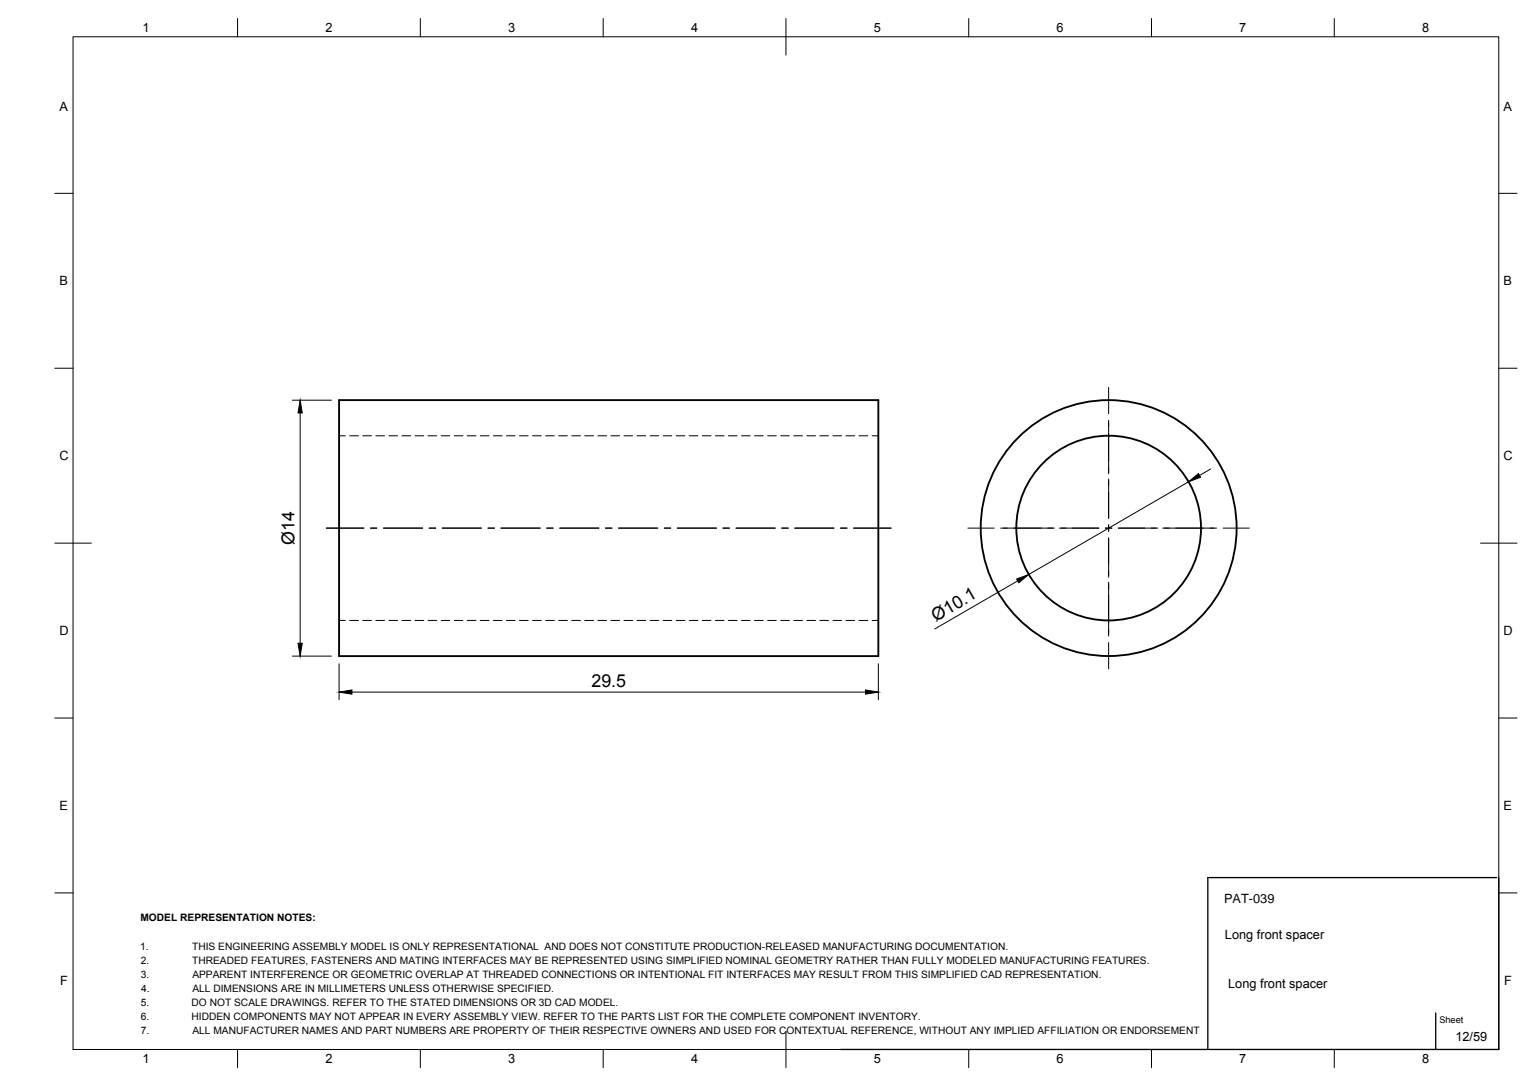
ISO-10303-21;
HEADER;
/* Generated by software containing ST-Developer
 * from STEP Tools, Inc. (www.steptools.com) 
 */

FILE_DESCRIPTION(
/* description */ ('Four-bar parallelogram arm'),
/* implementation_level */ '2;1');

FILE_NAME(
/* name */ 'Long front spacer.step',
/* time_stamp */ '2026-10-28T03:24:55-07:00',
/* author */ (''),
/* organization */ (''),
/* preprocessor_version */ 'ST-DEVELOPER v20.2',
/* originating_system */ 'Autodesk Translation Framework v15.17.0.0',
/* authorisation */ '');

FILE_SCHEMA (('AUTOMOTIVE_DESIGN { 1 0 10303 214 3 1 1 }'));
ENDSEC;

DATA;
#10=MECHANICAL_DESIGN_GEOMETRIC_PRESENTATION_REPRESENTATION('',(#629),#14512);
#529=SHAPE_REPRESENTATION_RELATIONSHIP('SRR','None',#14750,#579);
#579=ADVANCED_BREP_SHAPE_REPRESENTATION('',(#687),#14465);
#629=STYLED_ITEM('',(#15073),#687);
#687=MANIFOLD_SOLID_BREP('Body1',#7333);
#781=FACE_BOUND('',#1736,.T.);
#782=FACE_BOUND('',#1738,.T.);
#1044=PLANE('',#8076);
#1045=PLANE('',#8077);
#1267=FACE_OUTER_BOUND('',#1733,.T.);
#1268=FACE_OUTER_BOUND('',#1734,.T.);
#1269=FACE_OUTER_BOUND('',#1735,.T.);
#1270=FACE_OUTER_BOUND('',#1737,.T.);
#1733=EDGE_LOOP('',(#5276,#5277,#5278,#5279));
#1734=EDGE_LOOP('',(#5280,#5281,#5282,#5283));
#1735=EDGE_LOOP('',(#5284));
#1736=EDGE_LOOP('',(#5285));
#1737=EDGE_LOOP('',(#5286));
#1738=EDGE_LOOP('',(#5287));
#2400=LINE('',#11748,#2794);
#2401=LINE('',#11754,#2795);
#2794=VECTOR('',#9326,0.505);
#2795=VECTOR('',#9333,0.7);
#3156=CIRCLE('',#8071,0.505);
#3157=CIRCLE('',#8072,0.505);
#3158=CIRCLE('',#8074,0.7);
#3159=CIRCLE('',#8075,0.7);
#3641=VERTEX_POINT('',#11745);
#3642=VERTEX_POINT('',#11747);
#3643=VERTEX_POINT('',#11751);
#3644=VERTEX_POINT('',#11753);
#4269=EDGE_CURVE('',#3641,#3641,#3156,.T.);
#4270=EDGE_CURVE('',#3641,#3642,#2400,.T.);
#4271=EDGE_CURVE('',#3642,#3642,#3157,.T.);
#4272=EDGE_CURVE('',#3643,#3643,#3158,.T.);
#4273=EDGE_CURVE('',#3643,#3644,#2401,.T.);
#4274=EDGE_CURVE('',#3644,#3644,#3159,.T.);
#5276=ORIENTED_EDGE('',*,*,#4269,.F.);
#5277=ORIENTED_EDGE('',*,*,#4270,.T.);
#5278=ORIENTED_EDGE('',*,*,#4271,.T.);
#5279=ORIENTED_EDGE('',*,*,#4270,.F.);
#5280=ORIENTED_EDGE('',*,*,#4272,.F.);
#5281=ORIENTED_EDGE('',*,*,#4273,.T.);
#5282=ORIENTED_EDGE('',*,*,#4274,.T.);
#5283=ORIENTED_EDGE('',*,*,#4273,.F.);
#5284=ORIENTED_EDGE('',*,*,#4272,.T.);
#5285=ORIENTED_EDGE('',*,*,#4269,.T.);
#5286=ORIENTED_EDGE('',*,*,#4274,.F.);
#5287=ORIENTED_EDGE('',*,*,#4271,.F.);
#6742=CYLINDRICAL_SURFACE('',#8070,0.505);
#6743=CYLINDRICAL_SURFACE('',#8073,0.7);
#6972=ADVANCED_FACE('',(#1267),#6742,.F.);
#6973=ADVANCED_FACE('',(#1268),#6743,.T.);
#6974=ADVANCED_FACE('',(#1269,#781),#1044,.T.);
#6975=ADVANCED_FACE('',(#1270,#782),#1045,.F.);
#7333=CLOSED_SHELL('',(#6972,#6973,#6974,#6975));
#8069=AXIS2_PLACEMENT_3D('',#11743,#9320,#9321);
#8070=AXIS2_PLACEMENT_3D('',#11744,#9322,#9323);
#8071=AXIS2_PLACEMENT_3D('',#11746,#9324,#9325);
#8072=AXIS2_PLACEMENT_3D('',#11749,#9327,#9328);
#8073=AXIS2_PLACEMENT_3D('',#11750,#9329,#9330);
#8074=AXIS2_PLACEMENT_3D('',#11752,#9331,#9332);
#8075=AXIS2_PLACEMENT_3D('',#11755,#9334,#9335);
#8076=AXIS2_PLACEMENT_3D('',#11756,#9336,#9337);
#8077=AXIS2_PLACEMENT_3D('',#11757,#9338,#9339);
#9320=DIRECTION('axis',(0.,0.,1.));
#9321=DIRECTION('refdir',(1.,0.,0.));
#9322=DIRECTION('center_axis',(0.,1.,0.));
#9323=DIRECTION('ref_axis',(1.,0.,0.));
#9324=DIRECTION('center_axis',(0.,-1.,0.));
#9325=DIRECTION('ref_axis',(1.,0.,0.));
#9326=DIRECTION('',(0.,-1.,0.));
#9327=DIRECTION('center_axis',(0.,-1.,0.));
#9328=DIRECTION('ref_axis',(1.,0.,0.));
#9329=DIRECTION('center_axis',(0.,1.,0.));
#9330=DIRECTION('ref_axis',(1.,0.,0.));
#9331=DIRECTION('center_axis',(0.,1.,0.));
#9332=DIRECTION('ref_axis',(1.,0.,0.));
#9333=DIRECTION('',(0.,-1.,0.));
#9334=DIRECTION('center_axis',(0.,1.,0.));
#9335=DIRECTION('ref_axis',(1.,0.,0.));
#9336=DIRECTION('center_axis',(0.,1.,0.));
#9337=DIRECTION('ref_axis',(1.,0.,0.));
#9338=DIRECTION('center_axis',(0.,1.,0.));
#9339=DIRECTION('ref_axis',(1.,0.,0.));
#11743=CARTESIAN_POINT('',(0.,0.,0.));
#11744=CARTESIAN_POINT('Origin',(0.,-4.,8.));
#11745=CARTESIAN_POINT('',(-0.505,-1.05,8.));
#11746=CARTESIAN_POINT('Origin',(0.,-1.05,8.));
#11747=CARTESIAN_POINT('',(-0.505,-4.,8.));
#11748=CARTESIAN_POINT('',(-0.505,-4.,8.));
#11749=CARTESIAN_POINT('Origin',(0.,-4.,8.));
#11750=CARTESIAN_POINT('Origin',(0.,-4.,8.));
#11751=CARTESIAN_POINT('',(-0.7,-1.05,8.));
#11752=CARTESIAN_POINT('Origin',(0.,-1.05,8.));
#11753=CARTESIAN_POINT('',(-0.7,-4.,8.));
#11754=CARTESIAN_POINT('',(-0.7,-4.,8.));
#11755=CARTESIAN_POINT('Origin',(0.,-4.,8.));
#11756=CARTESIAN_POINT('Origin',(0.,-1.05,8.));
#11757=CARTESIAN_POINT('Origin',(0.,-4.,8.));
#14408=UNCERTAINTY_MEASURE_WITH_UNIT(LENGTH_MEASURE(0.001),#14513,
'DISTANCE_ACCURACY_VALUE',
'Maximum model space distance between geometric entities at asserted c
onnectivities');
#14455=UNCERTAINTY_MEASURE_WITH_UNIT(LENGTH_MEASURE(0.001),#14513,
'DISTANCE_ACCURACY_VALUE',
'Maximum model space distance between geometric entities at asserted c
onnectivities');
#14465=(
GEOMETRIC_REPRESENTATION_CONTEXT(3)
GLOBAL_UNCERTAINTY_ASSIGNED_CONTEXT((#14408))
GLOBAL_UNIT_ASSIGNED_CONTEXT((#14513,#14515,#14516))
REPRESENTATION_CONTEXT('','3D')
);
#14512=(
GEOMETRIC_REPRESENTATION_CONTEXT(3)
GLOBAL_UNCERTAINTY_ASSIGNED_CONTEXT((#14455))
GLOBAL_UNIT_ASSIGNED_CONTEXT((#14513,#14515,#14516))
REPRESENTATION_CONTEXT('','3D')
);
#14513=(
LENGTH_UNIT()
NAMED_UNIT(*)
SI_UNIT(.CENTI.,.METRE.)
);
#14515=(
NAMED_UNIT(*)
PLANE_ANGLE_UNIT()
SI_UNIT($,.RADIAN.)
);
#14516=(
NAMED_UNIT(*)
SI_UNIT($,.STERADIAN.)
SOLID_ANGLE_UNIT()
);
#14526=SHAPE_DEFINITION_REPRESENTATION(#14582,#14750);
#14582=PRODUCT_DEFINITION_SHAPE('',$,#14807);
#14750=SHAPE_REPRESENTATION('',(#8069),#14465);
#14797=PRODUCT_DEFINITION_CONTEXT('part definition',#14967,'design');
#14807=PRODUCT_DEFINITION('Long front spacer','Long front spacer',#14863,
#14797);
#14863=PRODUCT_DEFINITION_FORMATION('',$,#14978);
#14967=APPLICATION_CONTEXT(
'Core Data for Automotive Mechanical Design Process');
#14968=PRODUCT_CONTEXT('part definition',#14967,'mechanical');
#14978=PRODUCT('Long front spacer','Long front spacer',
'Long front spacer',(#14968));
#15067=COLOUR_RGB('Light Blue',0.38,0.62,0.78);
#15068=FILL_AREA_STYLE_COLOUR('',#15067);
#15069=FILL_AREA_STYLE('',(#15068));
#15070=SURFACE_STYLE_FILL_AREA(#15069);
#15071=SURFACE_SIDE_STYLE('',(#15070));
#15072=SURFACE_STYLE_USAGE(.BOTH.,#15071);
#15073=PRESENTATION_STYLE_ASSIGNMENT((#15072));
ENDSEC;
END-ISO-10303-21;
